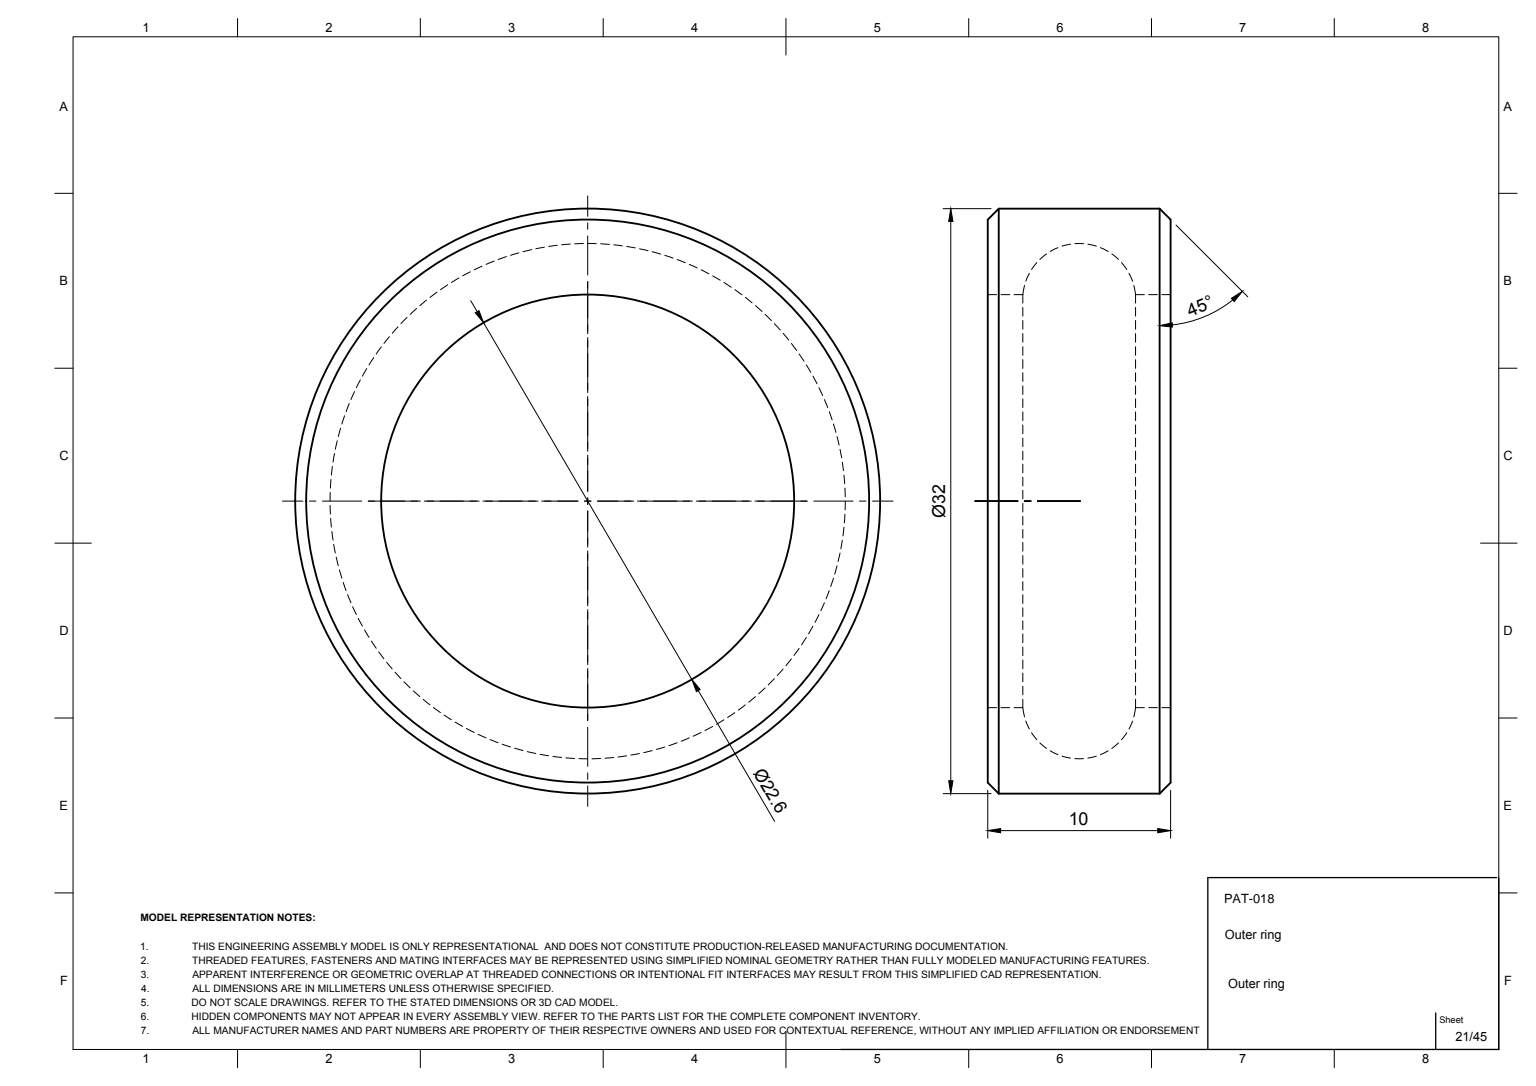
ISO-10303-21;
HEADER;
/* Generated by software containing ST-Developer
 * from STEP Tools, Inc. (www.steptools.com) 
 */

FILE_DESCRIPTION(
/* description */ ('Cam-driven reciprocating slide'),
/* implementation_level */ '2;1');

FILE_NAME(
/* name */ 'Outer ring.step',
/* time_stamp */ '2026-10-28T03:25:20-07:00',
/* author */ (''),
/* organization */ (''),
/* preprocessor_version */ 'ST-DEVELOPER v20.2',
/* originating_system */ 'Autodesk Translation Framework v15.17.0.0',
/* authorisation */ '');

FILE_SCHEMA (('AUTOMOTIVE_DESIGN { 1 0 10303 214 3 1 1 }'));
ENDSEC;

DATA;
#10=MECHANICAL_DESIGN_GEOMETRIC_PRESENTATION_REPRESENTATION('',(#436),#13277);
#317=CONICAL_SURFACE('',#7187,1.57,0.785398163397449);
#318=CONICAL_SURFACE('',#7191,1.57,0.785398163397449);
#331=TOROIDAL_SURFACE('',#7176,1.1,0.309556);
#362=SHAPE_REPRESENTATION_RELATIONSHIP('SRR','None',#13456,#399);
#399=ADVANCED_BREP_SHAPE_REPRESENTATION('',(#480),#13251);
#436=STYLED_ITEM('',(#13720),#480);
#480=MANIFOLD_SOLID_BREP('Body1',#6412);
#620=FACE_BOUND('',#1555,.T.);
#621=FACE_BOUND('',#1560,.T.);
#766=PLANE('',#7184);
#767=PLANE('',#7193);
#1060=FACE_OUTER_BOUND('',#1552,.T.);
#1061=FACE_OUTER_BOUND('',#1553,.T.);
#1062=FACE_OUTER_BOUND('',#1554,.T.);
#1063=FACE_OUTER_BOUND('',#1556,.T.);
#1064=FACE_OUTER_BOUND('',#1557,.T.);
#1065=FACE_OUTER_BOUND('',#1558,.T.);
#1066=FACE_OUTER_BOUND('',#1559,.T.);
#1067=FACE_OUTER_BOUND('',#1561,.T.);
#1552=EDGE_LOOP('',(#5040,#5041,#5042,#5043,#5044,#5045));
#1553=EDGE_LOOP('',(#5046,#5047,#5048,#5049,#5050));
#1554=EDGE_LOOP('',(#5051));
#1555=EDGE_LOOP('',(#5052));
#1556=EDGE_LOOP('',(#5053,#5054,#5055,#5056));
#1557=EDGE_LOOP('',(#5057,#5058,#5059,#5060));
#1558=EDGE_LOOP('',(#5061,#5062,#5063,#5064));
#1559=EDGE_LOOP('',(#5065));
#1560=EDGE_LOOP('',(#5066));
#1561=EDGE_LOOP('',(#5067,#5068,#5069,#5070,#5071));
#2037=LINE('',#11878,#2476);
#2038=LINE('',#11887,#2477);
#2039=LINE('',#11891,#2478);
#2040=LINE('',#11895,#2479);
#2041=LINE('',#11898,#2480);
#2476=VECTOR('',#8535,1.129765);
#2477=VECTOR('',#8546,1.57);
#2478=VECTOR('',#8551,1.6);
#2479=VECTOR('',#8556,1.57);
#2480=VECTOR('',#8561,1.129765);
#2858=CIRCLE('',#7177,1.129765);
#2859=CIRCLE('',#7178,1.129765);
#2860=CIRCLE('',#7179,0.309556);
#2861=CIRCLE('',#7180,1.129765);
#2862=CIRCLE('',#7181,1.129765);
#2863=CIRCLE('',#7183,1.129765);
#2864=CIRCLE('',#7185,1.54);
#2865=CIRCLE('',#7186,1.129765);
#2866=CIRCLE('',#7188,1.6);
#2867=CIRCLE('',#7190,1.6);
#2868=CIRCLE('',#7192,1.54);
#3269=VERTEX_POINT('',#11866);
#3270=VERTEX_POINT('',#11867);
#3271=VERTEX_POINT('',#11870);
#3272=VERTEX_POINT('',#11872);
#3273=VERTEX_POINT('',#11876);
#3274=VERTEX_POINT('',#11880);
#3275=VERTEX_POINT('',#11882);
#3276=VERTEX_POINT('',#11885);
#3277=VERTEX_POINT('',#11889);
#3278=VERTEX_POINT('',#11893);
#3910=EDGE_CURVE('',#3269,#3270,#2858,.T.);
#3911=EDGE_CURVE('',#3270,#3269,#2859,.T.);
#3912=EDGE_CURVE('',#3270,#3271,#2860,.T.);
#3913=EDGE_CURVE('',#3272,#3271,#2861,.T.);
#3914=EDGE_CURVE('',#3271,#3272,#2862,.T.);
#3915=EDGE_CURVE('',#3273,#3273,#2863,.T.);
#3916=EDGE_CURVE('',#3273,#3272,#2037,.T.);
#3917=EDGE_CURVE('',#3274,#3274,#2864,.T.);
#3918=EDGE_CURVE('',#3275,#3275,#2865,.T.);
#3919=EDGE_CURVE('',#3276,#3276,#2866,.T.);
#3920=EDGE_CURVE('',#3276,#3274,#2038,.T.);
#3921=EDGE_CURVE('',#3277,#3277,#2867,.T.);
#3922=EDGE_CURVE('',#3277,#3276,#2039,.T.);
#3923=EDGE_CURVE('',#3278,#3278,#2868,.T.);
#3924=EDGE_CURVE('',#3278,#3277,#2040,.T.);
#3925=EDGE_CURVE('',#3269,#3275,#2041,.T.);
#5040=ORIENTED_EDGE('',*,*,#3910,.F.);
#5041=ORIENTED_EDGE('',*,*,#3911,.F.);
#5042=ORIENTED_EDGE('',*,*,#3912,.T.);
#5043=ORIENTED_EDGE('',*,*,#3913,.F.);
#5044=ORIENTED_EDGE('',*,*,#3914,.F.);
#5045=ORIENTED_EDGE('',*,*,#3912,.F.);
#5046=ORIENTED_EDGE('',*,*,#3915,.T.);
#5047=ORIENTED_EDGE('',*,*,#3916,.T.);
#5048=ORIENTED_EDGE('',*,*,#3913,.T.);
#5049=ORIENTED_EDGE('',*,*,#3914,.T.);
#5050=ORIENTED_EDGE('',*,*,#3916,.F.);
#5051=ORIENTED_EDGE('',*,*,#3917,.F.);
#5052=ORIENTED_EDGE('',*,*,#3918,.T.);
#5053=ORIENTED_EDGE('',*,*,#3919,.F.);
#5054=ORIENTED_EDGE('',*,*,#3920,.T.);
#5055=ORIENTED_EDGE('',*,*,#3917,.T.);
#5056=ORIENTED_EDGE('',*,*,#3920,.F.);
#5057=ORIENTED_EDGE('',*,*,#3921,.F.);
#5058=ORIENTED_EDGE('',*,*,#3922,.T.);
#5059=ORIENTED_EDGE('',*,*,#3919,.T.);
#5060=ORIENTED_EDGE('',*,*,#3922,.F.);
#5061=ORIENTED_EDGE('',*,*,#3923,.F.);
#5062=ORIENTED_EDGE('',*,*,#3924,.T.);
#5063=ORIENTED_EDGE('',*,*,#3921,.T.);
#5064=ORIENTED_EDGE('',*,*,#3924,.F.);
#5065=ORIENTED_EDGE('',*,*,#3923,.T.);
#5066=ORIENTED_EDGE('',*,*,#3915,.F.);
#5067=ORIENTED_EDGE('',*,*,#3910,.T.);
#5068=ORIENTED_EDGE('',*,*,#3911,.T.);
#5069=ORIENTED_EDGE('',*,*,#3925,.T.);
#5070=ORIENTED_EDGE('',*,*,#3918,.F.);
#5071=ORIENTED_EDGE('',*,*,#3925,.F.);
#5962=CYLINDRICAL_SURFACE('',#7182,1.129765);
#5963=CYLINDRICAL_SURFACE('',#7189,1.6);
#5964=CYLINDRICAL_SURFACE('',#7194,1.129765);
#6178=ADVANCED_FACE('',(#1060),#331,.F.);
#6179=ADVANCED_FACE('',(#1061),#5962,.F.);
#6180=ADVANCED_FACE('',(#1062,#620),#766,.T.);
#6181=ADVANCED_FACE('',(#1063),#317,.T.);
#6182=ADVANCED_FACE('',(#1064),#5963,.T.);
#6183=ADVANCED_FACE('',(#1065),#318,.T.);
#6184=ADVANCED_FACE('',(#1066,#621),#767,.T.);
#6185=ADVANCED_FACE('',(#1067),#5964,.F.);
#6412=CLOSED_SHELL('',(#6178,#6179,#6180,#6181,#6182,#6183,#6184,#6185));
#7175=AXIS2_PLACEMENT_3D('',#11864,#8517,#8518);
#7176=AXIS2_PLACEMENT_3D('',#11865,#8519,#8520);
#7177=AXIS2_PLACEMENT_3D('',#11868,#8521,#8522);
#7178=AXIS2_PLACEMENT_3D('',#11869,#8523,#8524);
#7179=AXIS2_PLACEMENT_3D('',#11871,#8525,#8526);
#7180=AXIS2_PLACEMENT_3D('',#11873,#8527,#8528);
#7181=AXIS2_PLACEMENT_3D('',#11874,#8529,#8530);
#7182=AXIS2_PLACEMENT_3D('',#11875,#8531,#8532);
#7183=AXIS2_PLACEMENT_3D('',#11877,#8533,#8534);
#7184=AXIS2_PLACEMENT_3D('',#11879,#8536,#8537);
#7185=AXIS2_PLACEMENT_3D('',#11881,#8538,#8539);
#7186=AXIS2_PLACEMENT_3D('',#11883,#8540,#8541);
#7187=AXIS2_PLACEMENT_3D('',#11884,#8542,#8543);
#7188=AXIS2_PLACEMENT_3D('',#11886,#8544,#8545);
#7189=AXIS2_PLACEMENT_3D('',#11888,#8547,#8548);
#7190=AXIS2_PLACEMENT_3D('',#11890,#8549,#8550);
#7191=AXIS2_PLACEMENT_3D('',#11892,#8552,#8553);
#7192=AXIS2_PLACEMENT_3D('',#11894,#8554,#8555);
#7193=AXIS2_PLACEMENT_3D('',#11896,#8557,#8558);
#7194=AXIS2_PLACEMENT_3D('',#11897,#8559,#8560);
#8517=DIRECTION('axis',(0.,0.,1.));
#8518=DIRECTION('refdir',(1.,0.,0.));
#8519=DIRECTION('center_axis',(0.,-1.,0.));
#8520=DIRECTION('ref_axis',(0.,0.,-1.));
#8521=DIRECTION('center_axis',(0.,-1.,0.));
#8522=DIRECTION('ref_axis',(1.,0.,0.));
#8523=DIRECTION('center_axis',(0.,-1.,0.));
#8524=DIRECTION('ref_axis',(1.,0.,0.));
#8525=DIRECTION('center_axis',(1.,0.,1.22464679914735E-16));
#8526=DIRECTION('ref_axis',(-1.22464679914735E-16,0.,1.));
#8527=DIRECTION('center_axis',(0.,1.,0.));
#8528=DIRECTION('ref_axis',(1.,0.,0.));
#8529=DIRECTION('center_axis',(0.,1.,0.));
#8530=DIRECTION('ref_axis',(1.,0.,0.));
#8531=DIRECTION('center_axis',(0.,-1.,0.));
#8532=DIRECTION('ref_axis',(1.,0.,0.));
#8533=DIRECTION('center_axis',(0.,-1.,0.));
#8534=DIRECTION('ref_axis',(1.,0.,0.));
#8535=DIRECTION('',(0.,1.,0.));
#8536=DIRECTION('center_axis',(0.,1.,0.));
#8537=DIRECTION('ref_axis',(0.,0.,1.));
#8538=DIRECTION('center_axis',(0.,-1.,0.));
#8539=DIRECTION('ref_axis',(1.,0.,0.));
#8540=DIRECTION('center_axis',(0.,-1.,0.));
#8541=DIRECTION('ref_axis',(1.,0.,0.));
#8542=DIRECTION('center_axis',(0.,-1.,0.));
#8543=DIRECTION('ref_axis',(1.,0.,0.));
#8544=DIRECTION('center_axis',(0.,-1.,0.));
#8545=DIRECTION('ref_axis',(1.,0.,0.));
#8546=DIRECTION('',(0.707106781186548,0.707106781186547,8.65956056235494E-17));
#8547=DIRECTION('center_axis',(0.,-1.,0.));
#8548=DIRECTION('ref_axis',(1.,0.,0.));
#8549=DIRECTION('center_axis',(0.,-1.,0.));
#8550=DIRECTION('ref_axis',(1.,0.,0.));
#8551=DIRECTION('',(0.,1.,0.));
#8552=DIRECTION('center_axis',(0.,1.,0.));
#8553=DIRECTION('ref_axis',(1.,0.,0.));
#8554=DIRECTION('center_axis',(0.,-1.,0.));
#8555=DIRECTION('ref_axis',(1.,0.,0.));
#8556=DIRECTION('',(-0.707106781186548,0.707106781186547,-8.65956056235494E-17));
#8557=DIRECTION('center_axis',(0.,-1.,0.));
#8558=DIRECTION('ref_axis',(0.,0.,-1.));
#8559=DIRECTION('center_axis',(0.,-1.,0.));
#8560=DIRECTION('ref_axis',(1.,0.,0.));
#8561=DIRECTION('',(0.,1.,0.));
#11864=CARTESIAN_POINT('',(0.,0.,0.));
#11865=CARTESIAN_POINT('Origin',(0.,0.,0.));
#11866=CARTESIAN_POINT('',(-1.129765,0.308121667383195,-1.38356309103871E-16));
#11867=CARTESIAN_POINT('',(-1.38356309103871E-16,0.308121667383195,1.129765));
#11868=CARTESIAN_POINT('Origin',(0.,0.308121667383195,0.));
#11869=CARTESIAN_POINT('Origin',(0.,0.308121667383195,0.));
#11870=CARTESIAN_POINT('',(-1.38356309103871E-16,-0.308121667383195,1.129765));
#11871=CARTESIAN_POINT('Origin',(-1.34711147906209E-16,0.,1.1));
#11872=CARTESIAN_POINT('',(-1.129765,-0.308121667383195,1.38356309103871E-16));
#11873=CARTESIAN_POINT('Origin',(0.,-0.308121667383195,0.));
#11874=CARTESIAN_POINT('Origin',(0.,-0.308121667383195,0.));
#11875=CARTESIAN_POINT('Origin',(0.,0.,0.));
#11876=CARTESIAN_POINT('',(-1.129765,-0.5,-1.38356309103871E-16));
#11877=CARTESIAN_POINT('Origin',(0.,-0.5,0.));
#11878=CARTESIAN_POINT('',(-1.129765,0.,-1.38356309103871E-16));
#11879=CARTESIAN_POINT('Origin',(1.54,0.5,0.));
#11880=CARTESIAN_POINT('',(-1.54,0.5,-1.88595607068692E-16));
#11881=CARTESIAN_POINT('Origin',(0.,0.5,0.));
#11882=CARTESIAN_POINT('',(-1.129765,0.5,-1.38356309103871E-16));
#11883=CARTESIAN_POINT('Origin',(0.,0.5,0.));
#11884=CARTESIAN_POINT('Origin',(0.,0.47,0.));
#11885=CARTESIAN_POINT('',(-1.6,0.44,-1.95943487863577E-16));
#11886=CARTESIAN_POINT('Origin',(0.,0.44,0.));
#11887=CARTESIAN_POINT('',(-1.57,0.47,-1.92269547466134E-16));
#11888=CARTESIAN_POINT('Origin',(0.,0.,0.));
#11889=CARTESIAN_POINT('',(-1.6,-0.44,-1.95943487863577E-16));
#11890=CARTESIAN_POINT('Origin',(0.,-0.44,0.));
#11891=CARTESIAN_POINT('',(-1.6,0.,-1.95943487863577E-16));
#11892=CARTESIAN_POINT('Origin',(0.,-0.47,0.));
#11893=CARTESIAN_POINT('',(-1.54,-0.5,-1.88595607068692E-16));
#11894=CARTESIAN_POINT('Origin',(0.,-0.5,0.));
#11895=CARTESIAN_POINT('',(-1.57,-0.47,-1.92269547466134E-16));
#11896=CARTESIAN_POINT('Origin',(1.129765,-0.5,0.));
#11897=CARTESIAN_POINT('Origin',(0.,0.,0.));
#11898=CARTESIAN_POINT('',(-1.129765,0.,-1.38356309103871E-16));
#13207=UNCERTAINTY_MEASURE_WITH_UNIT(LENGTH_MEASURE(0.001),#13278,
'DISTANCE_ACCURACY_VALUE',
'Maximum model space distance between geometric entities at asserted c
onnectivities');
#13233=UNCERTAINTY_MEASURE_WITH_UNIT(LENGTH_MEASURE(0.001),#13278,
'DISTANCE_ACCURACY_VALUE',
'Maximum model space distance between geometric entities at asserted c
onnectivities');
#13251=(
GEOMETRIC_REPRESENTATION_CONTEXT(3)
GLOBAL_UNCERTAINTY_ASSIGNED_CONTEXT((#13207))
GLOBAL_UNIT_ASSIGNED_CONTEXT((#13278,#13280,#13281))
REPRESENTATION_CONTEXT('','3D')
);
#13277=(
GEOMETRIC_REPRESENTATION_CONTEXT(3)
GLOBAL_UNCERTAINTY_ASSIGNED_CONTEXT((#13233))
GLOBAL_UNIT_ASSIGNED_CONTEXT((#13278,#13280,#13281))
REPRESENTATION_CONTEXT('','3D')
);
#13278=(
LENGTH_UNIT()
NAMED_UNIT(*)
SI_UNIT(.CENTI.,.METRE.)
);
#13280=(
NAMED_UNIT(*)
PLANE_ANGLE_UNIT()
SI_UNIT($,.RADIAN.)
);
#13281=(
NAMED_UNIT(*)
SI_UNIT($,.STERADIAN.)
SOLID_ANGLE_UNIT()
);
#13299=SHAPE_DEFINITION_REPRESENTATION(#13342,#13456);
#13342=PRODUCT_DEFINITION_SHAPE('',$,#13500);
#13456=SHAPE_REPRESENTATION('',(#7175),#13251);
#13482=PRODUCT_DEFINITION_CONTEXT('part definition',#13613,'design');
#13500=PRODUCT_DEFINITION('Outer ring','Outer ring',#13543,#13482);
#13543=PRODUCT_DEFINITION_FORMATION('',$,#13632);
#13613=APPLICATION_CONTEXT(
'Core Data for Automotive Mechanical Design Process');
#13614=PRODUCT_CONTEXT('part definition',#13613,'mechanical');
#13632=PRODUCT('Outer ring','Outer ring','Outer ring',(#13614));
#13714=COLOUR_RGB('Grey',0.48,0.52,0.57);
#13715=FILL_AREA_STYLE_COLOUR('',#13714);
#13716=FILL_AREA_STYLE('',(#13715));
#13717=SURFACE_STYLE_FILL_AREA(#13716);
#13718=SURFACE_SIDE_STYLE('',(#13717));
#13719=SURFACE_STYLE_USAGE(.BOTH.,#13718);
#13720=PRESENTATION_STYLE_ASSIGNMENT((#13719));
ENDSEC;
END-ISO-10303-21;
